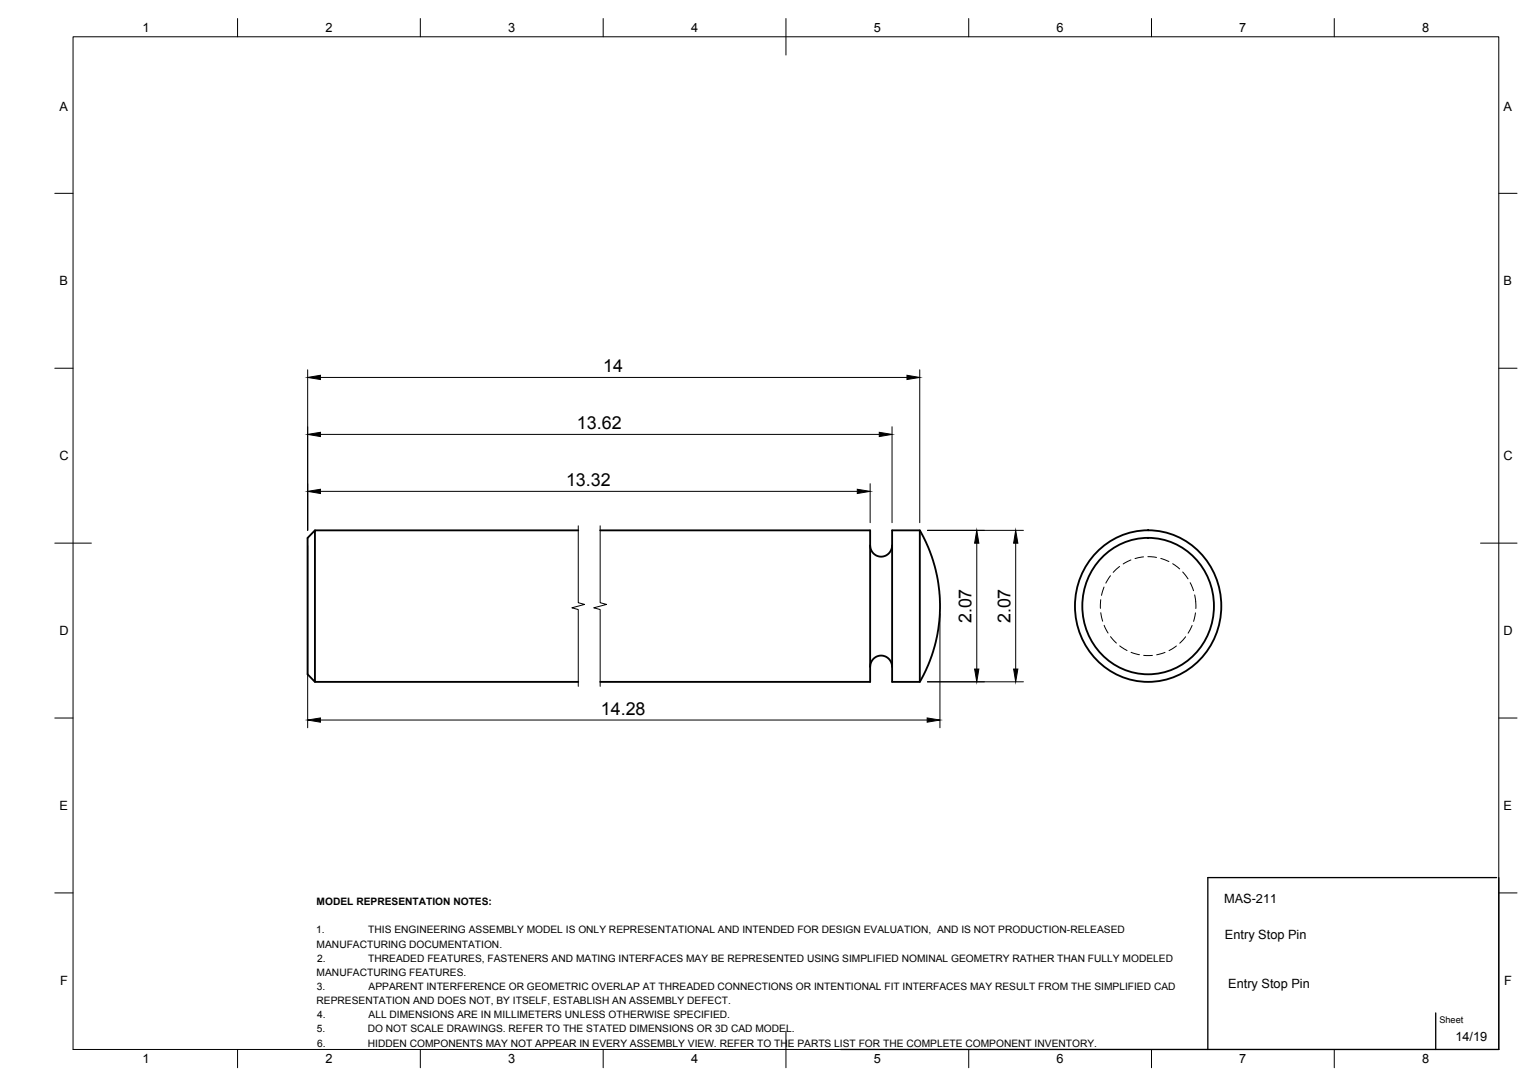
ISO-10303-21;
HEADER;
FILE_DESCRIPTION(
 (''),
 '2;1');
FILE_NAME ( 'Entry Stop Pin.step', '2026-10-05T20:07:59+06:00', ( '' ), ( '' ), 'STEP AP214', 'Unspecified', '' );
FILE_SCHEMA (('AUTOMOTIVE_DESIGN { 1 0 10303 214 3 1 1 }'));
ENDSEC;
DATA;
#10=MECHANICAL_DESIGN_GEOMETRIC_PRESENTATION_REPRESENTATION('',(#332),#196741);
#25=(
BOUNDED_CURVE()
B_SPLINE_CURVE(2,(#154494,#154495,#154496,#154497,#154498,#154499,#154500,
#154501,#154502),.UNSPECIFIED.,.F.,.F.)
B_SPLINE_CURVE_WITH_KNOTS((3,2,2,2,3),(1.42918797785348,1.62618617063892,
1.86180561965816,2.09742506867739,2.29442326146283),.UNSPECIFIED.)
CURVE()
GEOMETRIC_REPRESENTATION_ITEM()
RATIONAL_B_SPLINE_CURVE((1.,1.,1.,0.707106781186548,1.,0.707106781186548,
1.,1.,1.))
REPRESENTATION_ITEM('')
) ;
#51=(
BOUNDED_SURFACE()
B_SPLINE_SURFACE(2,2,((#154360,#154361,#154362),(#154363,#154364,#154365),
(#154366,#154367,#154368),(#154369,#154370,#154371),(#154372,#154373,#154374),
(#154375,#154376,#154377),(#154378,#154379,#154380),(#154381,#154382,#154383),
(#154384,#154385,#154386)),.UNSPECIFIED.,.T.,.F.,.F.)
B_SPLINE_SURFACE_WITH_KNOTS((3,2,2,2,3),(3,3),(0.,1.5707963267949,3.1415926535898,
4.71238898038469,6.28318530717959),(0.,1.05013832301181),.UNSPECIFIED.)
GEOMETRIC_REPRESENTATION_ITEM()
RATIONAL_B_SPLINE_SURFACE(((1.,0.963886720506905,1.),(0.707106781186548,
0.681570836366095,0.707106781186548),(1.,0.963886720506905,1.),(0.707106781186548,
0.681570836366095,0.707106781186548),(1.,0.963886720506905,1.),(0.707106781186548,
0.681570836366095,0.707106781186548),(1.,0.963886720506905,1.),(0.707106781186548,
0.681570836366095,0.707106781186548),(1.,0.963886720506905,1.)))
REPRESENTATION_ITEM('')
SURFACE()
) ;
#52=(
BOUNDED_SURFACE()
B_SPLINE_SURFACE(2,1,((#154391,#154392),(#154393,#154394),(#154395,#154396),
(#154397,#154398),(#154399,#154400),(#154401,#154402),(#154403,#154404),
(#154405,#154406),(#154407,#154408)),.UNSPECIFIED.,.T.,.F.,.F.)
B_SPLINE_SURFACE_WITH_KNOTS((3,2,2,2,3),(2,2),(0.,1.5707963267949,3.1415926535898,
4.71238898038469,6.28318530717959),(0.,0.0454859585810007),
 .UNSPECIFIED.)
GEOMETRIC_REPRESENTATION_ITEM()
RATIONAL_B_SPLINE_SURFACE(((1.,1.),(0.707106781186548,0.707106781186548),
(1.,1.),(0.707106781186548,0.707106781186548),(1.,1.),(0.707106781186548,
0.707106781186548),(1.,1.),(0.707106781186548,0.707106781186548),(1.,1.)))
REPRESENTATION_ITEM('')
SURFACE()
) ;
#53=(
BOUNDED_SURFACE()
B_SPLINE_SURFACE(2,2,((#154412,#154413,#154414,#154415,#154416,#154417,
#154418,#154419,#154420),(#154421,#154422,#154423,#154424,#154425,#154426,
#154427,#154428,#154429),(#154430,#154431,#154432,#154433,#154434,#154435,
#154436,#154437,#154438),(#154439,#154440,#154441,#154442,#154443,#154444,
#154445,#154446,#154447),(#154448,#154449,#154450,#154451,#154452,#154453,
#154454,#154455,#154456),(#154457,#154458,#154459,#154460,#154461,#154462,
#154463,#154464,#154465),(#154466,#154467,#154468,#154469,#154470,#154471,
#154472,#154473,#154474),(#154475,#154476,#154477,#154478,#154479,#154480,
#154481,#154482,#154483),(#154484,#154485,#154486,#154487,#154488,#154489,
#154490,#154491,#154492)),.UNSPECIFIED.,.T.,.F.,.F.)
B_SPLINE_SURFACE_WITH_KNOTS((3,2,2,2,3),(3,2,2,2,3),(0.,1.5707963267949,
3.1415926535898,4.71238898038469,6.28318530717959),(1.42918797785348,1.62618617063892,
1.86180561965816,2.09742506867739,2.29442326146283),.UNSPECIFIED.)
GEOMETRIC_REPRESENTATION_ITEM()
RATIONAL_B_SPLINE_SURFACE(((1.,1.,1.,0.707106781186548,1.,0.707106781186548,
1.,1.,1.),(0.707106781186548,0.707106781186548,0.707106781186548,0.5,0.707106781186548,
0.5,0.707106781186548,0.707106781186548,0.707106781186548),(1.,1.,1.,0.707106781186548,
1.,0.707106781186548,1.,1.,1.),(0.707106781186548,0.707106781186548,0.707106781186548,
0.5,0.707106781186548,0.5,0.707106781186548,0.707106781186548,0.707106781186548),
(1.,1.,1.,0.707106781186548,1.,0.707106781186548,1.,1.,1.),(0.707106781186548,
0.707106781186548,0.707106781186548,0.5,0.707106781186548,0.5,0.707106781186548,
0.707106781186548,0.707106781186548),(1.,1.,1.,0.707106781186548,1.,0.707106781186548,
1.,1.,1.),(0.707106781186548,0.707106781186548,0.707106781186548,0.5,0.707106781186548,
0.5,0.707106781186548,0.707106781186548,0.707106781186548),(1.,1.,1.,0.707106781186548,
1.,0.707106781186548,1.,1.,1.)))
REPRESENTATION_ITEM('')
SURFACE()
) ;
#54=(
BOUNDED_SURFACE()
B_SPLINE_SURFACE(2,1,((#154504,#154505),(#154506,#154507),(#154508,#154509),
(#154510,#154511),(#154512,#154513),(#154514,#154515),(#154516,#154517),
(#154518,#154519),(#154520,#154521)),.UNSPECIFIED.,.T.,.F.,.F.)
B_SPLINE_SURFACE_WITH_KNOTS((3,2,2,2,3),(2,2),(0.,1.5707963267949,3.1415926535898,
4.71238898038469,6.28318530717959),(0.,1.586514041419),.UNSPECIFIED.)
GEOMETRIC_REPRESENTATION_ITEM()
RATIONAL_B_SPLINE_SURFACE(((1.,1.),(0.707106781186548,0.707106781186548),
(1.,1.),(0.707106781186548,0.707106781186548),(1.,1.),(0.707106781186548,
0.707106781186548),(1.,1.),(0.707106781186548,0.707106781186548),(1.,1.)))
REPRESENTATION_ITEM('')
SURFACE()
) ;
#55=(
BOUNDED_SURFACE()
B_SPLINE_SURFACE(2,1,((#154525,#154526),(#154527,#154528),(#154529,#154530),
(#154531,#154532),(#154533,#154534),(#154535,#154536),(#154537,#154538),
(#154539,#154540),(#154541,#154542)),.UNSPECIFIED.,.T.,.F.,.F.)
B_SPLINE_SURFACE_WITH_KNOTS((3,2,2,2,3),(2,2),(0.,1.5707963267949,3.1415926535898,
4.71238898038469,6.28318530717959),(15.5153736066212,15.6567949628585),
 .UNSPECIFIED.)
GEOMETRIC_REPRESENTATION_ITEM()
RATIONAL_B_SPLINE_SURFACE(((1.,1.),(0.707106781186548,0.707106781186548),
(1.,1.),(0.707106781186548,0.707106781186548),(1.,1.),(0.707106781186548,
0.707106781186548),(1.,1.),(0.707106781186548,0.707106781186548),(1.,1.)))
REPRESENTATION_ITEM('')
SURFACE()
) ;
#165=ELLIPSE('',#9009,0.932157550311777,0.900000000000004) ;
#166=ELLIPSE('',#9011,1.03573061145752,0.999999999999994) ;
#167=ELLIPSE('',#9012,1.03573061145752,0.999999999999994) ;
#168=ELLIPSE('',#9013,1.03573061145752,0.999999999999994) ;
#169=ELLIPSE('',#9014,1.03573061145752,0.999999999999994) ;
#332=STYLED_ITEM('',(#196765),#351) ;
#351=MANIFOLD_SOLID_BREP('Entry Stop Pin',#8728) ;
#404=PLANE('',#9008) ;
#709=CIRCLE('',#9010,1.94783572104088) ;
#1054=FACE_OUTER_BOUND('',#1563,.T.) ;
#1055=FACE_OUTER_BOUND('',#1564,.T.) ;
#1056=FACE_OUTER_BOUND('',#1565,.T.) ;
#1057=FACE_OUTER_BOUND('',#1566,.T.) ;
#1058=FACE_OUTER_BOUND('',#1567,.T.) ;
#1059=FACE_OUTER_BOUND('',#1568,.T.) ;
#1563=EDGE_LOOP('',(#6552,#6553,#6554)) ;
#1564=EDGE_LOOP('',(#6555,#6556,#6557)) ;
#1565=EDGE_LOOP('',(#6558,#6559,#6560,#6561)) ;
#1566=EDGE_LOOP('',(#6562,#6563,#6564,#6565)) ;
#1567=EDGE_LOOP('',(#6566,#6567,#6568,#6569)) ;
#1568=EDGE_LOOP('',(#6570,#6571,#6572,#6573)) ;
#2044=LINE('',#154359,#2747) ;
#2045=LINE('',#154410,#2748) ;
#2046=LINE('',#154523,#2749) ;
#2047=LINE('',#154543,#2750) ;
#2747=VECTOR('',#10164,10.) ;
#2748=VECTOR('',#10169,10.) ;
#2749=VECTOR('',#10174,10.) ;
#2750=VECTOR('',#10177,10.) ;
#3770=VERTEX_POINT('',#154356) ;
#3771=VERTEX_POINT('',#154358) ;
#3772=VERTEX_POINT('',#154387) ;
#3773=VERTEX_POINT('',#154388) ;
#3774=VERTEX_POINT('',#154409) ;
#3775=VERTEX_POINT('',#154493) ;
#3776=VERTEX_POINT('',#154522) ;
#4784=EDGE_CURVE('',#3770,#3770,#165,.T.) ;
#4785=EDGE_CURVE('',#3770,#3771,#2044,.T.) ;
#4786=EDGE_CURVE('',#3772,#3773,#709,.T.) ;
#4787=EDGE_CURVE('',#3773,#3773,#166,.T.) ;
#4788=EDGE_CURVE('',#3773,#3774,#2045,.T.) ;
#4789=EDGE_CURVE('',#3774,#3774,#167,.T.) ;
#4790=EDGE_CURVE('',#3774,#3775,#25,.T.) ;
#4791=EDGE_CURVE('',#3775,#3775,#168,.T.) ;
#4792=EDGE_CURVE('',#3775,#3776,#2046,.T.) ;
#4793=EDGE_CURVE('',#3776,#3776,#169,.T.) ;
#4794=EDGE_CURVE('',#3776,#3770,#2047,.T.) ;
#6552=ORIENTED_EDGE('',*,*,#4784,.T.) ;
#6553=ORIENTED_EDGE('',*,*,#4785,.T.) ;
#6554=ORIENTED_EDGE('',*,*,#4785,.F.) ;
#6555=ORIENTED_EDGE('',*,*,#4786,.F.) ;
#6556=ORIENTED_EDGE('',*,*,#4786,.T.) ;
#6557=ORIENTED_EDGE('',*,*,#4787,.F.) ;
#6558=ORIENTED_EDGE('',*,*,#4788,.F.) ;
#6559=ORIENTED_EDGE('',*,*,#4787,.T.) ;
#6560=ORIENTED_EDGE('',*,*,#4788,.T.) ;
#6561=ORIENTED_EDGE('',*,*,#4789,.F.) ;
#6562=ORIENTED_EDGE('',*,*,#4790,.F.) ;
#6563=ORIENTED_EDGE('',*,*,#4789,.T.) ;
#6564=ORIENTED_EDGE('',*,*,#4790,.T.) ;
#6565=ORIENTED_EDGE('',*,*,#4791,.F.) ;
#6566=ORIENTED_EDGE('',*,*,#4792,.F.) ;
#6567=ORIENTED_EDGE('',*,*,#4791,.T.) ;
#6568=ORIENTED_EDGE('',*,*,#4792,.T.) ;
#6569=ORIENTED_EDGE('',*,*,#4793,.F.) ;
#6570=ORIENTED_EDGE('',*,*,#4794,.F.) ;
#6571=ORIENTED_EDGE('',*,*,#4793,.T.) ;
#6572=ORIENTED_EDGE('',*,*,#4794,.T.) ;
#6573=ORIENTED_EDGE('',*,*,#4784,.F.) ;
#8437=ADVANCED_FACE('',(#1054),#404,.T.) ;
#8438=ADVANCED_FACE('',(#1055),#51,.T.) ;
#8439=ADVANCED_FACE('',(#1056),#52,.T.) ;
#8440=ADVANCED_FACE('',(#1057),#53,.T.) ;
#8441=ADVANCED_FACE('',(#1058),#54,.T.) ;
#8442=ADVANCED_FACE('',(#1059),#55,.T.) ;
#8728=CLOSED_SHELL('',(#8437,#8438,#8439,#8440,#8441,#8442)) ;
#9008=AXIS2_PLACEMENT_3D('',#154355,#10160,#10161) ;
#9009=AXIS2_PLACEMENT_3D('',#154357,#10162,#10163) ;
#9010=AXIS2_PLACEMENT_3D('',#154389,#10165,#10166) ;
#9011=AXIS2_PLACEMENT_3D('',#154390,#10167,#10168) ;
#9012=AXIS2_PLACEMENT_3D('',#154411,#10170,#10171) ;
#9013=AXIS2_PLACEMENT_3D('',#154503,#10172,#10173) ;
#9014=AXIS2_PLACEMENT_3D('',#154524,#10175,#10176) ;
#10160=DIRECTION('center_axis',(-7.50393630258175E-16,1.,-7.64952095823687E-16)) ;
#10161=DIRECTION('ref_axis',(0.,7.64952095823687E-16,1.)) ;
#10162=DIRECTION('center_axis',(-4.70706556975765E-19,1.,-2.40039210366457E-19)) ;
#10163=DIRECTION('ref_axis',(0.950103467612796,5.22096546399878E-19,0.311934930442457)) ;
#10164=DIRECTION('',(0.311934930442522,-4.9210731940036E-16,-0.950103467612775)) ;
#10165=DIRECTION('center_axis',(-0.950103467612774,8.85448435361195E-14,
-0.311934930442524)) ;
#10166=DIRECTION('ref_axis',(-0.160144373097325,-0.858155219939114,0.487773921255037)) ;
#10167=DIRECTION('center_axis',(-1.02409251240679E-16,1.,-1.31144614757413E-15)) ;
#10168=DIRECTION('ref_axis',(0.950103467612728,5.06385247542231E-16,0.311934930442666)) ;
#10169=DIRECTION('',(2.34317168834017E-14,1.,0.)) ;
#10170=DIRECTION('center_axis',(0.,1.,0.)) ;
#10171=DIRECTION('ref_axis',(0.950103467612728,0.,0.311934930442666)) ;
#10172=DIRECTION('center_axis',(-1.73521265163545E-15,1.,-8.84880545094921E-16)) ;
#10173=DIRECTION('ref_axis',(0.950103467612728,1.92465670864857E-15,0.311934930442666)) ;
#10174=DIRECTION('',(6.71796199601783E-16,1.,0.)) ;
#10175=DIRECTION('center_axis',(0.,1.,0.)) ;
#10176=DIRECTION('ref_axis',(0.950103467612751,0.,0.311934930442595)) ;
#10177=DIRECTION('',(0.220571304604853,0.707106781186509,-0.671824604777889)) ;
#154355=CARTESIAN_POINT('Origin',(-29.5339383493105,-0.00455472950331615,
111.201234636506)) ;
#154356=CARTESIAN_POINT('',(-30.095421224107,-0.00455472950331526,112.911420878209)) ;
#154357=CARTESIAN_POINT('Origin',(-29.8146797867088,-0.00455472950331526,
112.056327757358)) ;
#154358=CARTESIAN_POINT('',(-29.8146797867088,-0.00455472950331526,112.056327757358)) ;
#154359=CARTESIAN_POINT('',(-30.0954212241071,-0.00455472950331526,112.911420878209)) ;
#154360=CARTESIAN_POINT('Ctrl Pts',(-29.8146797867088,-14.2808450589491,
112.056327757358)) ;
#154361=CARTESIAN_POINT('Ctrl Pts',(-29.9825532383426,-14.2808450589491,
112.567643204753)) ;
#154362=CARTESIAN_POINT('Ctrl Pts',(-30.1266147171513,-14.0045547295033,
113.006431224971)) ;
#154363=CARTESIAN_POINT('Ctrl Pts',(-29.8146797867088,-14.2808450589491,
112.056327757358)) ;
#154364=CARTESIAN_POINT('Ctrl Pts',(-29.4529681773643,-14.2808450589491,
112.741514877461)) ;
#154365=CARTESIAN_POINT('Ctrl Pts',(-29.1425634716928,-14.0045547295033,
113.329511781213)) ;
#154366=CARTESIAN_POINT('Ctrl Pts',(-29.8146797867088,-14.2808450589491,
112.056327757358)) ;
#154367=CARTESIAN_POINT('Ctrl Pts',(-29.2850947257306,-14.2808450589491,
112.230199430066)) ;
#154368=CARTESIAN_POINT('Ctrl Pts',(-28.8306285412503,-14.0045547295033,
112.3794083136)) ;
#154369=CARTESIAN_POINT('Ctrl Pts',(-29.8146797867088,-14.2808450589491,
112.056327757358)) ;
#154370=CARTESIAN_POINT('Ctrl Pts',(-29.1172212740968,-14.2808450589491,
111.718883982671)) ;
#154371=CARTESIAN_POINT('Ctrl Pts',(-28.5186936108078,-14.0045547295033,
111.429304845987)) ;
#154372=CARTESIAN_POINT('Ctrl Pts',(-29.8146797867088,-14.2808450589491,
112.056327757358)) ;
#154373=CARTESIAN_POINT('Ctrl Pts',(-29.646806335075,-14.2808450589491,
111.545012309963)) ;
#154374=CARTESIAN_POINT('Ctrl Pts',(-29.5027448562663,-14.0045547295033,
111.106224289745)) ;
#154375=CARTESIAN_POINT('Ctrl Pts',(-29.8146797867088,-14.2808450589491,
112.056327757358)) ;
#154376=CARTESIAN_POINT('Ctrl Pts',(-30.1763913960532,-14.2808450589491,
111.371140637255)) ;
#154377=CARTESIAN_POINT('Ctrl Pts',(-30.4867961017248,-14.0045547295033,
110.783143733503)) ;
#154378=CARTESIAN_POINT('Ctrl Pts',(-29.8146797867088,-14.2808450589491,
112.056327757358)) ;
#154379=CARTESIAN_POINT('Ctrl Pts',(-30.344264847687,-14.2808450589491,
111.88245608465)) ;
#154380=CARTESIAN_POINT('Ctrl Pts',(-30.7987310321673,-14.0045547295033,
111.733247201116)) ;
#154381=CARTESIAN_POINT('Ctrl Pts',(-29.8146797867088,-14.2808450589491,
112.056327757358)) ;
#154382=CARTESIAN_POINT('Ctrl Pts',(-30.5121382993208,-14.2808450589491,
112.393771532045)) ;
#154383=CARTESIAN_POINT('Ctrl Pts',(-31.1106659626098,-14.0045547295033,
112.683350668729)) ;
#154384=CARTESIAN_POINT('Ctrl Pts',(-29.8146797867088,-14.2808450589491,
112.056327757358)) ;
#154385=CARTESIAN_POINT('Ctrl Pts',(-29.9825532383426,-14.2808450589491,
112.567643204753)) ;
#154386=CARTESIAN_POINT('Ctrl Pts',(-30.1266147171513,-14.0045547295033,
113.006431224971)) ;
#154387=CARTESIAN_POINT('',(-29.8146797867088,-14.2808450589491,112.056327757358)) ;
#154388=CARTESIAN_POINT('',(-30.1266147171513,-14.0045547295033,113.006431224971)) ;
#154389=CARTESIAN_POINT('Origin',(-29.8146797867086,-12.3330093379082,112.056327757358)) ;
#154390=CARTESIAN_POINT('Origin',(-29.8146797867088,-14.0045547295033,112.056327757358)) ;
#154391=CARTESIAN_POINT('Ctrl Pts',(-30.1266147171513,-14.0045547295033,
113.006431224971)) ;
#154392=CARTESIAN_POINT('Ctrl Pts',(-30.1266147171513,-13.5496951436933,
113.006431224971)) ;
#154393=CARTESIAN_POINT('Ctrl Pts',(-29.1425634716928,-14.0045547295033,
113.329511781213)) ;
#154394=CARTESIAN_POINT('Ctrl Pts',(-29.1425634716928,-13.5496951436933,
113.329511781213)) ;
#154395=CARTESIAN_POINT('Ctrl Pts',(-28.8306285412503,-14.0045547295033,
112.3794083136)) ;
#154396=CARTESIAN_POINT('Ctrl Pts',(-28.8306285412503,-13.5496951436933,
112.3794083136)) ;
#154397=CARTESIAN_POINT('Ctrl Pts',(-28.5186936108078,-14.0045547295033,
111.429304845987)) ;
#154398=CARTESIAN_POINT('Ctrl Pts',(-28.5186936108078,-13.5496951436933,
111.429304845987)) ;
#154399=CARTESIAN_POINT('Ctrl Pts',(-29.5027448562663,-14.0045547295033,
111.106224289745)) ;
#154400=CARTESIAN_POINT('Ctrl Pts',(-29.5027448562663,-13.5496951436933,
111.106224289745)) ;
#154401=CARTESIAN_POINT('Ctrl Pts',(-30.4867961017248,-14.0045547295033,
110.783143733503)) ;
#154402=CARTESIAN_POINT('Ctrl Pts',(-30.4867961017248,-13.5496951436933,
110.783143733503)) ;
#154403=CARTESIAN_POINT('Ctrl Pts',(-30.7987310321673,-14.0045547295033,
111.733247201116)) ;
#154404=CARTESIAN_POINT('Ctrl Pts',(-30.7987310321673,-13.5496951436933,
111.733247201116)) ;
#154405=CARTESIAN_POINT('Ctrl Pts',(-31.1106659626098,-14.0045547295033,
112.683350668729)) ;
#154406=CARTESIAN_POINT('Ctrl Pts',(-31.1106659626098,-13.5496951436933,
112.683350668729)) ;
#154407=CARTESIAN_POINT('Ctrl Pts',(-30.1266147171513,-14.0045547295033,
113.006431224971)) ;
#154408=CARTESIAN_POINT('Ctrl Pts',(-30.1266147171513,-13.5496951436933,
113.006431224971)) ;
#154409=CARTESIAN_POINT('',(-30.1266147171513,-13.6255050746616,113.006431224971)) ;
#154410=CARTESIAN_POINT('',(-30.1266147171513,-14.0045547295033,113.006431224971)) ;
#154411=CARTESIAN_POINT('Origin',(-29.8146797867088,-13.6255050746616,112.056327757358)) ;
#154412=CARTESIAN_POINT('Ctrl Pts',(-30.1266147171513,-13.6255050746616,
113.006431224971)) ;
#154413=CARTESIAN_POINT('Ctrl Pts',(-30.0958894083694,-13.6255050746616,
112.912846891931)) ;
#154414=CARTESIAN_POINT('Ctrl Pts',(-30.0651640995875,-13.6255050746616,
112.819262558892)) ;
#154415=CARTESIAN_POINT('Ctrl Pts',(-30.0183738600211,-13.6255050746616,
112.67674703875)) ;
#154416=CARTESIAN_POINT('Ctrl Pts',(-30.0183738600211,-13.4755050746616,
112.67674703875)) ;
#154417=CARTESIAN_POINT('Ctrl Pts',(-30.0183738600211,-13.3255050746616,
112.67674703875)) ;
#154418=CARTESIAN_POINT('Ctrl Pts',(-30.0651640995875,-13.3255050746616,
112.819262558892)) ;
#154419=CARTESIAN_POINT('Ctrl Pts',(-30.0958894083694,-13.3255050746616,
112.912846891931)) ;
#154420=CARTESIAN_POINT('Ctrl Pts',(-30.1266147171513,-13.3255050746616,
113.006431224971)) ;
#154421=CARTESIAN_POINT('Ctrl Pts',(-29.1425634716928,-13.6255050746616,
113.329511781213)) ;
#154422=CARTESIAN_POINT('Ctrl Pts',(-29.2087663213927,-13.6255050746616,
113.204104305322)) ;
#154423=CARTESIAN_POINT('Ctrl Pts',(-29.2749691710926,-13.6255050746616,
113.07869682943)) ;
#154424=CARTESIAN_POINT('Ctrl Pts',(-29.375786618345,-13.6255050746616,
112.887719225852)) ;
#154425=CARTESIAN_POINT('Ctrl Pts',(-29.375786618345,-13.4755050746616,
112.887719225852)) ;
#154426=CARTESIAN_POINT('Ctrl Pts',(-29.375786618345,-13.3255050746616,
112.887719225852)) ;
#154427=CARTESIAN_POINT('Ctrl Pts',(-29.2749691710926,-13.3255050746616,
113.07869682943)) ;
#154428=CARTESIAN_POINT('Ctrl Pts',(-29.2087663213927,-13.3255050746616,
113.204104305322)) ;
#154429=CARTESIAN_POINT('Ctrl Pts',(-29.1425634716928,-13.3255050746616,
113.329511781213)) ;
#154430=CARTESIAN_POINT('Ctrl Pts',(-28.8306285412503,-13.6255050746616,
112.3794083136)) ;
#154431=CARTESIAN_POINT('Ctrl Pts',(-28.9275566997321,-13.6255050746616,
112.347585170748)) ;
#154432=CARTESIAN_POINT('Ctrl Pts',(-29.0244848582139,-13.6255050746616,
112.315762027896)) ;
#154433=CARTESIAN_POINT('Ctrl Pts',(-29.1720925450327,-13.6255050746616,
112.26729994446)) ;
#154434=CARTESIAN_POINT('Ctrl Pts',(-29.1720925450326,-13.4755050746616,
112.26729994446)) ;
#154435=CARTESIAN_POINT('Ctrl Pts',(-29.1720925450327,-13.3255050746616,
112.26729994446)) ;
#154436=CARTESIAN_POINT('Ctrl Pts',(-29.0244848582139,-13.3255050746616,
112.315762027896)) ;
#154437=CARTESIAN_POINT('Ctrl Pts',(-28.9275566997321,-13.3255050746616,
112.347585170748)) ;
#154438=CARTESIAN_POINT('Ctrl Pts',(-28.8306285412503,-13.3255050746616,
112.3794083136)) ;
#154439=CARTESIAN_POINT('Ctrl Pts',(-28.5186936108078,-13.6255050746616,
111.429304845987)) ;
#154440=CARTESIAN_POINT('Ctrl Pts',(-28.6463470780715,-13.6255050746616,
111.491066036175)) ;
#154441=CARTESIAN_POINT('Ctrl Pts',(-28.7740005453352,-13.6255050746616,
111.552827226362)) ;
#154442=CARTESIAN_POINT('Ctrl Pts',(-28.9683984717204,-13.6255050746616,
111.646880663068)) ;
#154443=CARTESIAN_POINT('Ctrl Pts',(-28.9683984717203,-13.4755050746616,
111.646880663068)) ;
#154444=CARTESIAN_POINT('Ctrl Pts',(-28.9683984717204,-13.3255050746616,
111.646880663068)) ;
#154445=CARTESIAN_POINT('Ctrl Pts',(-28.7740005453352,-13.3255050746616,
111.552827226362)) ;
#154446=CARTESIAN_POINT('Ctrl Pts',(-28.6463470780715,-13.3255050746616,
111.491066036175)) ;
#154447=CARTESIAN_POINT('Ctrl Pts',(-28.5186936108078,-13.3255050746616,
111.429304845987)) ;
#154448=CARTESIAN_POINT('Ctrl Pts',(-29.5027448562663,-13.6255050746616,
111.106224289745)) ;
#154449=CARTESIAN_POINT('Ctrl Pts',(-29.5334701650482,-13.6255050746616,
111.199808622785)) ;
#154450=CARTESIAN_POINT('Ctrl Pts',(-29.5641954738301,-13.6255050746616,
111.293392955824)) ;
#154451=CARTESIAN_POINT('Ctrl Pts',(-29.6109857133965,-13.6255050746616,
111.435908475966)) ;
#154452=CARTESIAN_POINT('Ctrl Pts',(-29.6109857133965,-13.4755050746616,
111.435908475966)) ;
#154453=CARTESIAN_POINT('Ctrl Pts',(-29.6109857133965,-13.3255050746616,
111.435908475966)) ;
#154454=CARTESIAN_POINT('Ctrl Pts',(-29.5641954738301,-13.3255050746616,
111.293392955824)) ;
#154455=CARTESIAN_POINT('Ctrl Pts',(-29.5334701650482,-13.3255050746616,
111.199808622785)) ;
#154456=CARTESIAN_POINT('Ctrl Pts',(-29.5027448562663,-13.3255050746616,
111.106224289745)) ;
#154457=CARTESIAN_POINT('Ctrl Pts',(-30.4867961017248,-13.6255050746616,
110.783143733503)) ;
#154458=CARTESIAN_POINT('Ctrl Pts',(-30.4205932520249,-13.6255050746616,
110.908551209394)) ;
#154459=CARTESIAN_POINT('Ctrl Pts',(-30.354390402325,-13.6255050746616,
111.033958685286)) ;
#154460=CARTESIAN_POINT('Ctrl Pts',(-30.2535729550726,-13.6255050746616,
111.224936288864)) ;
#154461=CARTESIAN_POINT('Ctrl Pts',(-30.2535729550726,-13.4755050746616,
111.224936288864)) ;
#154462=CARTESIAN_POINT('Ctrl Pts',(-30.2535729550726,-13.3255050746616,
111.224936288864)) ;
#154463=CARTESIAN_POINT('Ctrl Pts',(-30.354390402325,-13.3255050746616,
111.033958685286)) ;
#154464=CARTESIAN_POINT('Ctrl Pts',(-30.4205932520249,-13.3255050746616,
110.908551209394)) ;
#154465=CARTESIAN_POINT('Ctrl Pts',(-30.4867961017248,-13.3255050746616,
110.783143733503)) ;
#154466=CARTESIAN_POINT('Ctrl Pts',(-30.7987310321673,-13.6255050746616,
111.733247201116)) ;
#154467=CARTESIAN_POINT('Ctrl Pts',(-30.7018028736855,-13.6255050746616,
111.765070343968)) ;
#154468=CARTESIAN_POINT('Ctrl Pts',(-30.6048747152037,-13.6255050746616,
111.79689348682)) ;
#154469=CARTESIAN_POINT('Ctrl Pts',(-30.4572670283849,-13.6255050746616,
111.845355570256)) ;
#154470=CARTESIAN_POINT('Ctrl Pts',(-30.4572670283849,-13.4755050746616,
111.845355570256)) ;
#154471=CARTESIAN_POINT('Ctrl Pts',(-30.4572670283849,-13.3255050746616,
111.845355570256)) ;
#154472=CARTESIAN_POINT('Ctrl Pts',(-30.6048747152037,-13.3255050746616,
111.79689348682)) ;
#154473=CARTESIAN_POINT('Ctrl Pts',(-30.7018028736855,-13.3255050746616,
111.765070343968)) ;
#154474=CARTESIAN_POINT('Ctrl Pts',(-30.7987310321673,-13.3255050746616,
111.733247201116)) ;
#154475=CARTESIAN_POINT('Ctrl Pts',(-31.1106659626098,-13.6255050746616,
112.683350668729)) ;
#154476=CARTESIAN_POINT('Ctrl Pts',(-30.9830124953461,-13.6255050746616,
112.621589478541)) ;
#154477=CARTESIAN_POINT('Ctrl Pts',(-30.8553590280824,-13.6255050746616,
112.559828288353)) ;
#154478=CARTESIAN_POINT('Ctrl Pts',(-30.6609611016972,-13.6255050746616,
112.465774851648)) ;
#154479=CARTESIAN_POINT('Ctrl Pts',(-30.6609611016972,-13.4755050746616,
112.465774851648)) ;
#154480=CARTESIAN_POINT('Ctrl Pts',(-30.6609611016972,-13.3255050746616,
112.465774851648)) ;
#154481=CARTESIAN_POINT('Ctrl Pts',(-30.8553590280824,-13.3255050746616,
112.559828288353)) ;
#154482=CARTESIAN_POINT('Ctrl Pts',(-30.9830124953461,-13.3255050746616,
112.621589478541)) ;
#154483=CARTESIAN_POINT('Ctrl Pts',(-31.1106659626098,-13.3255050746616,
112.683350668729)) ;
#154484=CARTESIAN_POINT('Ctrl Pts',(-30.1266147171513,-13.6255050746616,
113.006431224971)) ;
#154485=CARTESIAN_POINT('Ctrl Pts',(-30.0958894083694,-13.6255050746616,
112.912846891931)) ;
#154486=CARTESIAN_POINT('Ctrl Pts',(-30.0651640995875,-13.6255050746616,
112.819262558892)) ;
#154487=CARTESIAN_POINT('Ctrl Pts',(-30.0183738600211,-13.6255050746616,
112.67674703875)) ;
#154488=CARTESIAN_POINT('Ctrl Pts',(-30.0183738600211,-13.4755050746616,
112.67674703875)) ;
#154489=CARTESIAN_POINT('Ctrl Pts',(-30.0183738600211,-13.3255050746616,
112.67674703875)) ;
#154490=CARTESIAN_POINT('Ctrl Pts',(-30.0651640995875,-13.3255050746616,
112.819262558892)) ;
#154491=CARTESIAN_POINT('Ctrl Pts',(-30.0958894083694,-13.3255050746616,
112.912846891931)) ;
#154492=CARTESIAN_POINT('Ctrl Pts',(-30.1266147171513,-13.3255050746616,
113.006431224971)) ;
#154493=CARTESIAN_POINT('',(-30.1266147171513,-13.3255050746616,113.006431224971)) ;
#154494=CARTESIAN_POINT('Ctrl Pts',(-30.1266147171513,-13.6255050746616,
113.006431224971)) ;
#154495=CARTESIAN_POINT('Ctrl Pts',(-30.0958894083694,-13.6255050746616,
112.912846891931)) ;
#154496=CARTESIAN_POINT('Ctrl Pts',(-30.0651640995875,-13.6255050746616,
112.819262558892)) ;
#154497=CARTESIAN_POINT('Ctrl Pts',(-30.0183738600211,-13.6255050746616,
112.67674703875)) ;
#154498=CARTESIAN_POINT('Ctrl Pts',(-30.0183738600211,-13.4755050746616,
112.67674703875)) ;
#154499=CARTESIAN_POINT('Ctrl Pts',(-30.0183738600211,-13.3255050746616,
112.67674703875)) ;
#154500=CARTESIAN_POINT('Ctrl Pts',(-30.0651640995875,-13.3255050746616,
112.819262558892)) ;
#154501=CARTESIAN_POINT('Ctrl Pts',(-30.0958894083694,-13.3255050746616,
112.912846891931)) ;
#154502=CARTESIAN_POINT('Ctrl Pts',(-30.1266147171513,-13.3255050746616,
113.006431224971)) ;
#154503=CARTESIAN_POINT('Origin',(-29.8146797867088,-13.3255050746616,112.056327757358)) ;
#154504=CARTESIAN_POINT('Ctrl Pts',(-30.1266147171513,-13.3255050746616,
113.006431224971)) ;
#154505=CARTESIAN_POINT('Ctrl Pts',(-30.1266147171513,2.53963533952835,
113.006431224971)) ;
#154506=CARTESIAN_POINT('Ctrl Pts',(-29.1425634716928,-13.3255050746616,
113.329511781213)) ;
#154507=CARTESIAN_POINT('Ctrl Pts',(-29.1425634716928,2.53963533952835,
113.329511781213)) ;
#154508=CARTESIAN_POINT('Ctrl Pts',(-28.8306285412503,-13.3255050746616,
112.3794083136)) ;
#154509=CARTESIAN_POINT('Ctrl Pts',(-28.8306285412503,2.53963533952835,
112.3794083136)) ;
#154510=CARTESIAN_POINT('Ctrl Pts',(-28.5186936108078,-13.3255050746616,
111.429304845987)) ;
#154511=CARTESIAN_POINT('Ctrl Pts',(-28.5186936108078,2.53963533952835,
111.429304845987)) ;
#154512=CARTESIAN_POINT('Ctrl Pts',(-29.5027448562663,-13.3255050746616,
111.106224289745)) ;
#154513=CARTESIAN_POINT('Ctrl Pts',(-29.5027448562663,2.53963533952835,
111.106224289745)) ;
#154514=CARTESIAN_POINT('Ctrl Pts',(-30.4867961017248,-13.3255050746616,
110.783143733503)) ;
#154515=CARTESIAN_POINT('Ctrl Pts',(-30.4867961017248,2.53963533952835,
110.783143733503)) ;
#154516=CARTESIAN_POINT('Ctrl Pts',(-30.7987310321673,-13.3255050746616,
111.733247201116)) ;
#154517=CARTESIAN_POINT('Ctrl Pts',(-30.7987310321673,2.53963533952835,
111.733247201116)) ;
#154518=CARTESIAN_POINT('Ctrl Pts',(-31.1106659626098,-13.3255050746616,
112.683350668729)) ;
#154519=CARTESIAN_POINT('Ctrl Pts',(-31.1106659626098,2.53963533952835,
112.683350668729)) ;
#154520=CARTESIAN_POINT('Ctrl Pts',(-30.1266147171513,-13.3255050746616,
113.006431224971)) ;
#154521=CARTESIAN_POINT('Ctrl Pts',(-30.1266147171513,2.53963533952835,
113.006431224971)) ;
#154522=CARTESIAN_POINT('',(-30.1266147171513,-0.104554729503315,113.006431224971)) ;
#154523=CARTESIAN_POINT('',(-30.1266147171513,-13.3255050746616,113.006431224971)) ;
#154524=CARTESIAN_POINT('Origin',(-29.8146797867088,-0.104554729503315,
112.056327757358)) ;
#154525=CARTESIAN_POINT('Ctrl Pts',(-30.1266147171513,-0.104554729503315,
113.006431224971)) ;
#154526=CARTESIAN_POINT('Ctrl Pts',(-30.095421224107,-0.00455472950331526,
112.911420878209)) ;
#154527=CARTESIAN_POINT('Ctrl Pts',(-29.1425634716928,-0.104554729503315,
113.329511781213)) ;
#154528=CARTESIAN_POINT('Ctrl Pts',(-29.2097751031944,-0.00455472950331526,
113.202193378827)) ;
#154529=CARTESIAN_POINT('Ctrl Pts',(-28.8306285412503,-0.104554729503315,
112.3794083136)) ;
#154530=CARTESIAN_POINT('Ctrl Pts',(-28.9290336657961,-0.00455472950331526,
112.347100257976)) ;
#154531=CARTESIAN_POINT('Ctrl Pts',(-28.5186936108078,-0.104554729503315,
111.429304845987)) ;
#154532=CARTESIAN_POINT('Ctrl Pts',(-28.6482922283979,-0.00455472950331526,
111.492007137124)) ;
#154533=CARTESIAN_POINT('Ctrl Pts',(-29.5027448562663,-0.104554729503315,
111.106224289745)) ;
#154534=CARTESIAN_POINT('Ctrl Pts',(-29.5339383493105,-0.00455472950331526,
111.201234636506)) ;
#154535=CARTESIAN_POINT('Ctrl Pts',(-30.4867961017248,-0.104554729503315,
110.783143733503)) ;
#154536=CARTESIAN_POINT('Ctrl Pts',(-30.4195844702232,-0.00455472950331526,
110.910462135889)) ;
#154537=CARTESIAN_POINT('Ctrl Pts',(-30.7987310321673,-0.104554729503315,
111.733247201116)) ;
#154538=CARTESIAN_POINT('Ctrl Pts',(-30.7003259076214,-0.00455472950331526,
111.76555525674)) ;
#154539=CARTESIAN_POINT('Ctrl Pts',(-31.1106659626098,-0.104554729503315,
112.683350668729)) ;
#154540=CARTESIAN_POINT('Ctrl Pts',(-30.9810673450197,-0.00455472950331526,
112.620648377591)) ;
#154541=CARTESIAN_POINT('Ctrl Pts',(-30.1266147171513,-0.104554729503315,
113.006431224971)) ;
#154542=CARTESIAN_POINT('Ctrl Pts',(-30.095421224107,-0.00455472950331526,
112.911420878209)) ;
#154543=CARTESIAN_POINT('',(-30.1266147171513,-0.104554729503315,113.006431224971)) ;
#196737=UNCERTAINTY_MEASURE_WITH_UNIT(LENGTH_MEASURE(0.01),#196742,
'DISTANCE_ACCURACY_VALUE',
'Maximum model space distance between geometric entities at asserted c
onnectivities') ;
#196738=UNCERTAINTY_MEASURE_WITH_UNIT(LENGTH_MEASURE(0.01),#196742,
'DISTANCE_ACCURACY_VALUE',
'Maximum model space distance between geometric entities at asserted c
onnectivities') ;
#196740=(
GEOMETRIC_REPRESENTATION_CONTEXT(3)
GLOBAL_UNCERTAINTY_ASSIGNED_CONTEXT((#196737))
GLOBAL_UNIT_ASSIGNED_CONTEXT((#196742,#196744,#196745))
REPRESENTATION_CONTEXT('','3D')
) ;
#196741=(
GEOMETRIC_REPRESENTATION_CONTEXT(3)
GLOBAL_UNCERTAINTY_ASSIGNED_CONTEXT((#196738))
GLOBAL_UNIT_ASSIGNED_CONTEXT((#196742,#196744,#196745))
REPRESENTATION_CONTEXT('','3D')
) ;
#196742=(
LENGTH_UNIT()
NAMED_UNIT(*)
SI_UNIT(.MILLI.,.METRE.)
) ;
#196744=(
NAMED_UNIT(*)
PLANE_ANGLE_UNIT()
SI_UNIT($,.RADIAN.)
) ;
#196745=(
NAMED_UNIT(*)
SI_UNIT($,.STERADIAN.)
SOLID_ANGLE_UNIT()
) ;
#196753=PRODUCT_DEFINITION_CONTEXT('part definition',#196761,'design') ;
#196761=APPLICATION_CONTEXT(
'Core Data for Automotive Mechanical Design Process') ;
#196762=PRODUCT_CONTEXT('part definition',#196761,'mechanical') ;
#196765=PRESENTATION_STYLE_ASSIGNMENT((#196767)) ;
#196767=SURFACE_STYLE_USAGE(.BOTH.,#196769) ;
#196769=SURFACE_SIDE_STYLE('',(#196771)) ;
#196771=SURFACE_STYLE_FILL_AREA(#196773) ;
#196773=FILL_AREA_STYLE('Steel - Satin',(#196775)) ;
#196775=FILL_AREA_STYLE_COLOUR('Steel - Satin',#196777) ;
#196777=COLOUR_RGB('Steel - Satin', 0.09019608, 0.27058824, 0.51372549) ;
#197091=CARTESIAN_POINT ( '', ( 0.0, 0.0, 0.0 ) ) ;
#197092=DIRECTION ( '', ( 0.0, 0.0, 1.0 ) ) ;
#197093=DIRECTION ( '', ( 1.0, 0.0, 0.0 ) ) ;
#197094=AXIS2_PLACEMENT_3D ( '', #197091, #197092, #197093 ) ;
#197095=ADVANCED_BREP_SHAPE_REPRESENTATION ( 'Entry Stop Pin', ( #351, #197094, #197105, #197407 ), #196740 ) ;
#197096=PRODUCT( 'Entry Stop Pin', 'Entry Stop Pin', '', ( #196762 ) ) ;
#197097=PRODUCT_DEFINITION_FORMATION ( '', '', #197096 ) ;
#197098=PRODUCT_DEFINITION( 'Entry Stop Pin', 'Entry Stop Pin', #197097, #196753 ) ;
#197099=PRODUCT_DEFINITION_SHAPE ( '', '', #197098 ) ;
#197100=SHAPE_DEFINITION_REPRESENTATION ( #197099, #197095 ) ;
#197102=CARTESIAN_POINT ( '', ( 0.0, 0.0, 0.0 ) ) ;
#197103=DIRECTION ( '', ( 0.0, 0.0, 1.0 ) ) ;
#197104=DIRECTION ( '', ( 1.0, 0.0, 0.0 ) ) ;
#197105=AXIS2_PLACEMENT_3D ( '', #197102, #197103, #197104 ) ;
#197404=CARTESIAN_POINT ( '', ( 0.0, 0.0, 0.0 ) ) ;
#197405=DIRECTION ( '', ( 0.0, 0.0, 1.0 ) ) ;
#197406=DIRECTION ( '', ( 1.0, 0.0, 0.0 ) ) ;
#197407=AXIS2_PLACEMENT_3D ( '', #197404, #197405, #197406 ) ;
ENDSEC;
END-ISO-10303-21;
